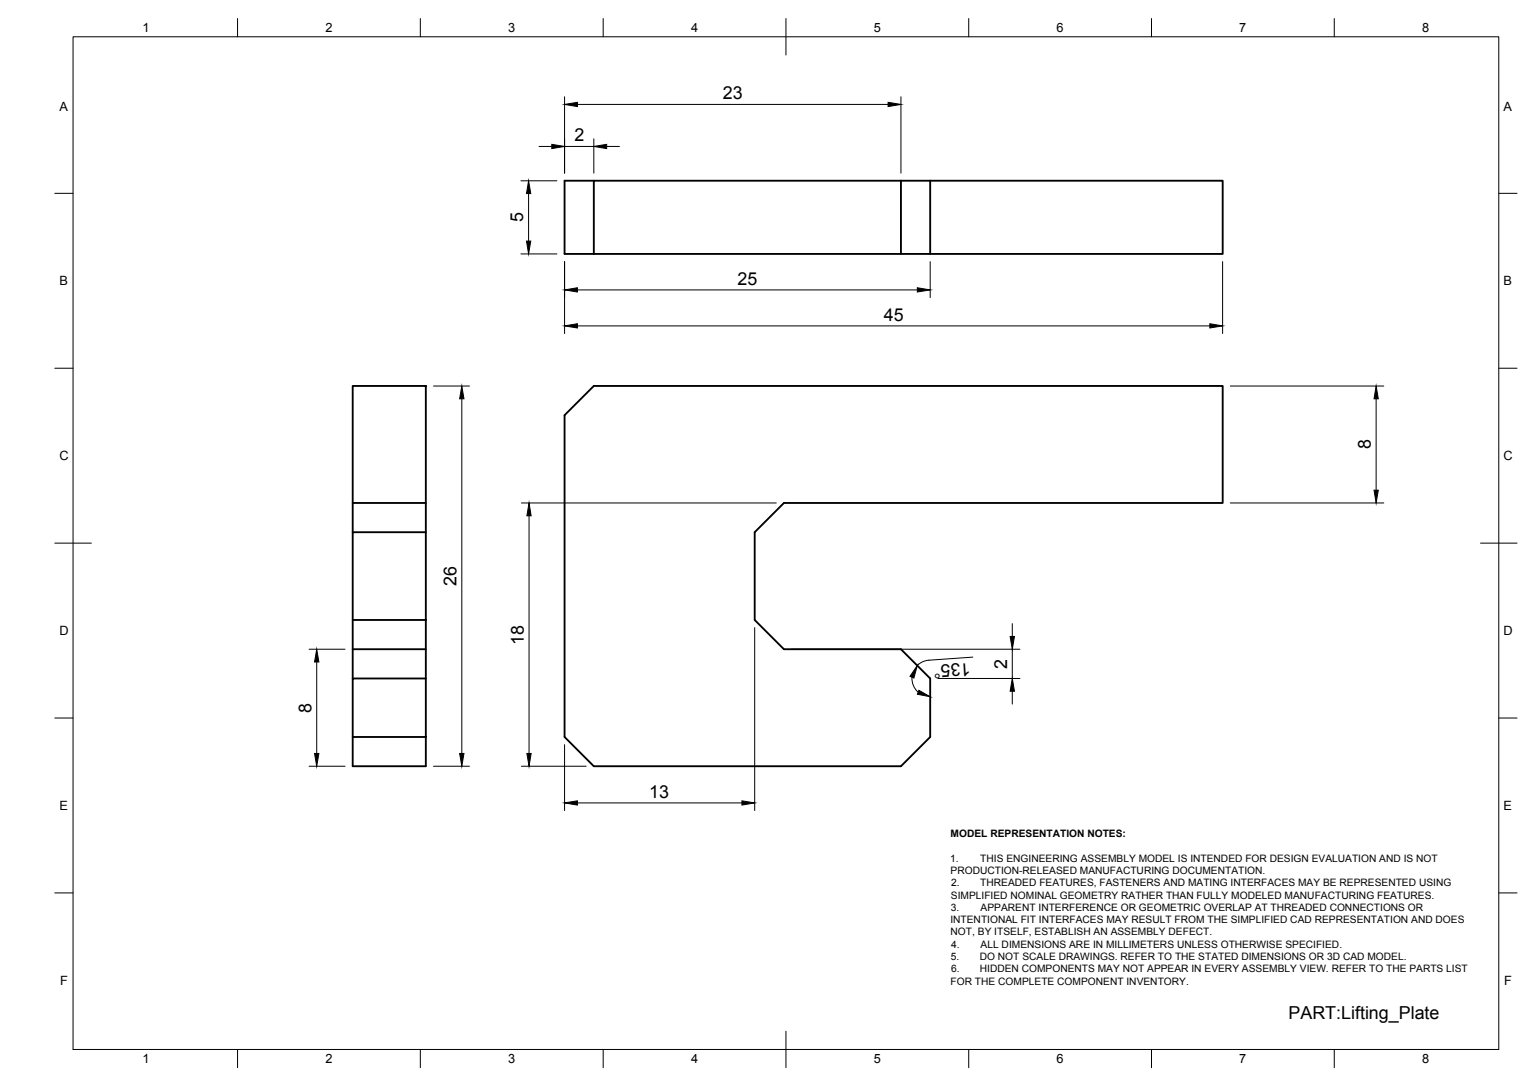
ISO-10303-21;
HEADER;
/* Generated by software containing ST-Developer
 * from STEP Tools, Inc. (www.steptools.com) 
 */

FILE_DESCRIPTION(
/* description */ ('STEP AP214'),
/* implementation_level */ '2;1');

FILE_NAME(
/* name */ 'Lifting_Plate.step',
/* time_stamp */ '2026-10-05T13:15:56-07:00',
/* author */ (''),
/* organization */ (''),
/* preprocessor_version */ 'ST-DEVELOPER v20.2',
/* originating_system */ 'Autodesk Translation Framework v15.15.0.0',
/* authorisation */ '');

FILE_SCHEMA (('AUTOMOTIVE_DESIGN { 1 0 10303 214 3 1 1 }'));
ENDSEC;

DATA;
#10=MECHANICAL_DESIGN_GEOMETRIC_PRESENTATION_REPRESENTATION('',(#1355),#37881);
#1331=SHAPE_REPRESENTATION_RELATIONSHIP('SRR','None',#37964,#1343);
#1343=ADVANCED_BREP_SHAPE_REPRESENTATION('',(#1367),#37879);
#1355=STYLED_ITEM('',(#38023),#1367);
#1367=MANIFOLD_SOLID_BREP('Body1',#10829);
#1547=PLANE('',#11824);
#1548=PLANE('',#11825);
#1549=PLANE('',#11826);
#1550=PLANE('',#11827);
#1551=PLANE('',#11828);
#1552=PLANE('',#11829);
#1553=PLANE('',#11830);
#1554=PLANE('',#11831);
#1555=PLANE('',#11832);
#1556=PLANE('',#11833);
#1557=PLANE('',#11834);
#1558=PLANE('',#11835);
#1559=PLANE('',#11836);
#1560=PLANE('',#11837);
#1561=PLANE('',#11838);
#1562=PLANE('',#11839);
#2154=FACE_OUTER_BOUND('',#2849,.T.);
#2155=FACE_OUTER_BOUND('',#2850,.T.);
#2156=FACE_OUTER_BOUND('',#2851,.T.);
#2157=FACE_OUTER_BOUND('',#2852,.T.);
#2158=FACE_OUTER_BOUND('',#2853,.T.);
#2159=FACE_OUTER_BOUND('',#2854,.T.);
#2160=FACE_OUTER_BOUND('',#2855,.T.);
#2161=FACE_OUTER_BOUND('',#2856,.T.);
#2162=FACE_OUTER_BOUND('',#2857,.T.);
#2163=FACE_OUTER_BOUND('',#2858,.T.);
#2164=FACE_OUTER_BOUND('',#2859,.T.);
#2165=FACE_OUTER_BOUND('',#2860,.T.);
#2166=FACE_OUTER_BOUND('',#2861,.T.);
#2167=FACE_OUTER_BOUND('',#2862,.T.);
#2168=FACE_OUTER_BOUND('',#2863,.T.);
#2169=FACE_OUTER_BOUND('',#2864,.T.);
#2849=EDGE_LOOP('',(#9933,#9934,#9935,#9936));
#2850=EDGE_LOOP('',(#9937,#9938,#9939,#9940));
#2851=EDGE_LOOP('',(#9941,#9942,#9943,#9944));
#2852=EDGE_LOOP('',(#9945,#9946,#9947,#9948));
#2853=EDGE_LOOP('',(#9949,#9950,#9951,#9952));
#2854=EDGE_LOOP('',(#9953,#9954,#9955,#9956));
#2855=EDGE_LOOP('',(#9957,#9958,#9959,#9960));
#2856=EDGE_LOOP('',(#9961,#9962,#9963,#9964));
#2857=EDGE_LOOP('',(#9965,#9966,#9967,#9968,#9969,#9970,#9971,#9972,#9973,
#9974,#9975,#9976,#9977,#9978));
#2858=EDGE_LOOP('',(#9979,#9980,#9981,#9982,#9983,#9984,#9985,#9986,#9987,
#9988,#9989,#9990,#9991,#9992));
#2859=EDGE_LOOP('',(#9993,#9994,#9995,#9996));
#2860=EDGE_LOOP('',(#9997,#9998,#9999,#10000));
#2861=EDGE_LOOP('',(#10001,#10002,#10003,#10004));
#2862=EDGE_LOOP('',(#10005,#10006,#10007,#10008));
#2863=EDGE_LOOP('',(#10009,#10010,#10011,#10012));
#2864=EDGE_LOOP('',(#10013,#10014,#10015,#10016));
#3128=LINE('',#37715,#3429);
#3129=LINE('',#37717,#3430);
#3130=LINE('',#37719,#3431);
#3131=LINE('',#37720,#3432);
#3132=LINE('',#37724,#3433);
#3133=LINE('',#37726,#3434);
#3134=LINE('',#37728,#3435);
#3135=LINE('',#37729,#3436);
#3136=LINE('',#37733,#3437);
#3137=LINE('',#37735,#3438);
#3138=LINE('',#37737,#3439);
#3139=LINE('',#37738,#3440);
#3140=LINE('',#37742,#3441);
#3141=LINE('',#37744,#3442);
#3142=LINE('',#37746,#3443);
#3143=LINE('',#37747,#3444);
#3144=LINE('',#37750,#3445);
#3145=LINE('',#37752,#3446);
#3146=LINE('',#37753,#3447);
#3147=LINE('',#37756,#3448);
#3148=LINE('',#37758,#3449);
#3149=LINE('',#37759,#3450);
#3150=LINE('',#37763,#3451);
#3151=LINE('',#37765,#3452);
#3152=LINE('',#37767,#3453);
#3153=LINE('',#37768,#3454);
#3154=LINE('',#37772,#3455);
#3155=LINE('',#37774,#3456);
#3156=LINE('',#37776,#3457);
#3157=LINE('',#37777,#3458);
#3158=LINE('',#37779,#3459);
#3159=LINE('',#37780,#3460);
#3160=LINE('',#37781,#3461);
#3161=LINE('',#37782,#3462);
#3162=LINE('',#37783,#3463);
#3163=LINE('',#37784,#3464);
#3164=LINE('',#37786,#3465);
#3165=LINE('',#37787,#3466);
#3166=LINE('',#37788,#3467);
#3167=LINE('',#37789,#3468);
#3168=LINE('',#37790,#3469);
#3169=LINE('',#37791,#3470);
#3429=VECTOR('',#13869,1000.);
#3430=VECTOR('',#13870,1000.);
#3431=VECTOR('',#13871,1000.);
#3432=VECTOR('',#13872,1000.);
#3433=VECTOR('',#13875,1000.);
#3434=VECTOR('',#13876,1000.);
#3435=VECTOR('',#13877,1000.);
#3436=VECTOR('',#13878,1000.);
#3437=VECTOR('',#13881,1000.);
#3438=VECTOR('',#13882,1000.);
#3439=VECTOR('',#13883,1000.);
#3440=VECTOR('',#13884,1000.);
#3441=VECTOR('',#13887,1000.);
#3442=VECTOR('',#13888,1000.);
#3443=VECTOR('',#13889,1000.);
#3444=VECTOR('',#13890,1000.);
#3445=VECTOR('',#13893,1000.);
#3446=VECTOR('',#13894,1000.);
#3447=VECTOR('',#13895,1000.);
#3448=VECTOR('',#13898,1000.);
#3449=VECTOR('',#13899,1000.);
#3450=VECTOR('',#13900,1000.);
#3451=VECTOR('',#13903,1000.);
#3452=VECTOR('',#13904,1000.);
#3453=VECTOR('',#13905,1000.);
#3454=VECTOR('',#13906,1000.);
#3455=VECTOR('',#13909,1000.);
#3456=VECTOR('',#13910,1000.);
#3457=VECTOR('',#13911,1000.);
#3458=VECTOR('',#13912,1000.);
#3459=VECTOR('',#13915,1000.);
#3460=VECTOR('',#13916,1000.);
#3461=VECTOR('',#13917,1000.);
#3462=VECTOR('',#13918,1000.);
#3463=VECTOR('',#13919,1000.);
#3464=VECTOR('',#13920,1000.);
#3465=VECTOR('',#13923,1000.);
#3466=VECTOR('',#13924,1000.);
#3467=VECTOR('',#13925,1000.);
#3468=VECTOR('',#13926,1000.);
#3469=VECTOR('',#13927,1000.);
#3470=VECTOR('',#13928,1000.);
#5041=VERTEX_POINT('',#37713);
#5042=VERTEX_POINT('',#37714);
#5043=VERTEX_POINT('',#37716);
#5044=VERTEX_POINT('',#37718);
#5045=VERTEX_POINT('',#37722);
#5046=VERTEX_POINT('',#37723);
#5047=VERTEX_POINT('',#37725);
#5048=VERTEX_POINT('',#37727);
#5049=VERTEX_POINT('',#37731);
#5050=VERTEX_POINT('',#37732);
#5051=VERTEX_POINT('',#37734);
#5052=VERTEX_POINT('',#37736);
#5053=VERTEX_POINT('',#37740);
#5054=VERTEX_POINT('',#37741);
#5055=VERTEX_POINT('',#37743);
#5056=VERTEX_POINT('',#37745);
#5057=VERTEX_POINT('',#37749);
#5058=VERTEX_POINT('',#37751);
#5059=VERTEX_POINT('',#37755);
#5060=VERTEX_POINT('',#37757);
#5061=VERTEX_POINT('',#37761);
#5062=VERTEX_POINT('',#37762);
#5063=VERTEX_POINT('',#37764);
#5064=VERTEX_POINT('',#37766);
#5065=VERTEX_POINT('',#37770);
#5066=VERTEX_POINT('',#37771);
#5067=VERTEX_POINT('',#37773);
#5068=VERTEX_POINT('',#37775);
#6677=EDGE_CURVE('',#5041,#5042,#3128,.T.);
#6678=EDGE_CURVE('',#5042,#5043,#3129,.T.);
#6679=EDGE_CURVE('',#5044,#5043,#3130,.T.);
#6680=EDGE_CURVE('',#5044,#5041,#3131,.T.);
#6681=EDGE_CURVE('',#5045,#5046,#3132,.T.);
#6682=EDGE_CURVE('',#5045,#5047,#3133,.T.);
#6683=EDGE_CURVE('',#5047,#5048,#3134,.T.);
#6684=EDGE_CURVE('',#5048,#5046,#3135,.T.);
#6685=EDGE_CURVE('',#5049,#5050,#3136,.T.);
#6686=EDGE_CURVE('',#5049,#5051,#3137,.T.);
#6687=EDGE_CURVE('',#5051,#5052,#3138,.T.);
#6688=EDGE_CURVE('',#5052,#5050,#3139,.T.);
#6689=EDGE_CURVE('',#5053,#5054,#3140,.T.);
#6690=EDGE_CURVE('',#5054,#5055,#3141,.T.);
#6691=EDGE_CURVE('',#5056,#5055,#3142,.T.);
#6692=EDGE_CURVE('',#5053,#5056,#3143,.T.);
#6693=EDGE_CURVE('',#5057,#5056,#3144,.T.);
#6694=EDGE_CURVE('',#5058,#5057,#3145,.T.);
#6695=EDGE_CURVE('',#5058,#5053,#3146,.T.);
#6696=EDGE_CURVE('',#5059,#5057,#3147,.T.);
#6697=EDGE_CURVE('',#5059,#5060,#3148,.T.);
#6698=EDGE_CURVE('',#5060,#5058,#3149,.T.);
#6699=EDGE_CURVE('',#5061,#5062,#3150,.T.);
#6700=EDGE_CURVE('',#5062,#5063,#3151,.T.);
#6701=EDGE_CURVE('',#5064,#5063,#3152,.T.);
#6702=EDGE_CURVE('',#5064,#5061,#3153,.T.);
#6703=EDGE_CURVE('',#5065,#5066,#3154,.T.);
#6704=EDGE_CURVE('',#5066,#5067,#3155,.T.);
#6705=EDGE_CURVE('',#5068,#5067,#3156,.T.);
#6706=EDGE_CURVE('',#5068,#5065,#3157,.T.);
#6707=EDGE_CURVE('',#5051,#5054,#3158,.T.);
#6708=EDGE_CURVE('',#5060,#5062,#3159,.T.);
#6709=EDGE_CURVE('',#5061,#5066,#3160,.T.);
#6710=EDGE_CURVE('',#5065,#5042,#3161,.T.);
#6711=EDGE_CURVE('',#5041,#5048,#3162,.T.);
#6712=EDGE_CURVE('',#5047,#5052,#3163,.T.);
#6713=EDGE_CURVE('',#5055,#5049,#3164,.T.);
#6714=EDGE_CURVE('',#5050,#5045,#3165,.T.);
#6715=EDGE_CURVE('',#5046,#5044,#3166,.T.);
#6716=EDGE_CURVE('',#5043,#5068,#3167,.T.);
#6717=EDGE_CURVE('',#5067,#5064,#3168,.T.);
#6718=EDGE_CURVE('',#5063,#5059,#3169,.T.);
#9933=ORIENTED_EDGE('',*,*,#6677,.T.);
#9934=ORIENTED_EDGE('',*,*,#6678,.T.);
#9935=ORIENTED_EDGE('',*,*,#6679,.F.);
#9936=ORIENTED_EDGE('',*,*,#6680,.T.);
#9937=ORIENTED_EDGE('',*,*,#6681,.F.);
#9938=ORIENTED_EDGE('',*,*,#6682,.T.);
#9939=ORIENTED_EDGE('',*,*,#6683,.T.);
#9940=ORIENTED_EDGE('',*,*,#6684,.T.);
#9941=ORIENTED_EDGE('',*,*,#6685,.F.);
#9942=ORIENTED_EDGE('',*,*,#6686,.T.);
#9943=ORIENTED_EDGE('',*,*,#6687,.T.);
#9944=ORIENTED_EDGE('',*,*,#6688,.T.);
#9945=ORIENTED_EDGE('',*,*,#6689,.T.);
#9946=ORIENTED_EDGE('',*,*,#6690,.T.);
#9947=ORIENTED_EDGE('',*,*,#6691,.F.);
#9948=ORIENTED_EDGE('',*,*,#6692,.F.);
#9949=ORIENTED_EDGE('',*,*,#6693,.F.);
#9950=ORIENTED_EDGE('',*,*,#6694,.F.);
#9951=ORIENTED_EDGE('',*,*,#6695,.T.);
#9952=ORIENTED_EDGE('',*,*,#6692,.T.);
#9953=ORIENTED_EDGE('',*,*,#6696,.F.);
#9954=ORIENTED_EDGE('',*,*,#6697,.T.);
#9955=ORIENTED_EDGE('',*,*,#6698,.T.);
#9956=ORIENTED_EDGE('',*,*,#6694,.T.);
#9957=ORIENTED_EDGE('',*,*,#6699,.T.);
#9958=ORIENTED_EDGE('',*,*,#6700,.T.);
#9959=ORIENTED_EDGE('',*,*,#6701,.F.);
#9960=ORIENTED_EDGE('',*,*,#6702,.T.);
#9961=ORIENTED_EDGE('',*,*,#6703,.T.);
#9962=ORIENTED_EDGE('',*,*,#6704,.T.);
#9963=ORIENTED_EDGE('',*,*,#6705,.F.);
#9964=ORIENTED_EDGE('',*,*,#6706,.T.);
#9965=ORIENTED_EDGE('',*,*,#6687,.F.);
#9966=ORIENTED_EDGE('',*,*,#6707,.T.);
#9967=ORIENTED_EDGE('',*,*,#6689,.F.);
#9968=ORIENTED_EDGE('',*,*,#6695,.F.);
#9969=ORIENTED_EDGE('',*,*,#6698,.F.);
#9970=ORIENTED_EDGE('',*,*,#6708,.T.);
#9971=ORIENTED_EDGE('',*,*,#6699,.F.);
#9972=ORIENTED_EDGE('',*,*,#6709,.T.);
#9973=ORIENTED_EDGE('',*,*,#6703,.F.);
#9974=ORIENTED_EDGE('',*,*,#6710,.T.);
#9975=ORIENTED_EDGE('',*,*,#6677,.F.);
#9976=ORIENTED_EDGE('',*,*,#6711,.T.);
#9977=ORIENTED_EDGE('',*,*,#6683,.F.);
#9978=ORIENTED_EDGE('',*,*,#6712,.T.);
#9979=ORIENTED_EDGE('',*,*,#6691,.T.);
#9980=ORIENTED_EDGE('',*,*,#6713,.T.);
#9981=ORIENTED_EDGE('',*,*,#6685,.T.);
#9982=ORIENTED_EDGE('',*,*,#6714,.T.);
#9983=ORIENTED_EDGE('',*,*,#6681,.T.);
#9984=ORIENTED_EDGE('',*,*,#6715,.T.);
#9985=ORIENTED_EDGE('',*,*,#6679,.T.);
#9986=ORIENTED_EDGE('',*,*,#6716,.T.);
#9987=ORIENTED_EDGE('',*,*,#6705,.T.);
#9988=ORIENTED_EDGE('',*,*,#6717,.T.);
#9989=ORIENTED_EDGE('',*,*,#6701,.T.);
#9990=ORIENTED_EDGE('',*,*,#6718,.T.);
#9991=ORIENTED_EDGE('',*,*,#6696,.T.);
#9992=ORIENTED_EDGE('',*,*,#6693,.T.);
#9993=ORIENTED_EDGE('',*,*,#6707,.F.);
#9994=ORIENTED_EDGE('',*,*,#6686,.F.);
#9995=ORIENTED_EDGE('',*,*,#6713,.F.);
#9996=ORIENTED_EDGE('',*,*,#6690,.F.);
#9997=ORIENTED_EDGE('',*,*,#6712,.F.);
#9998=ORIENTED_EDGE('',*,*,#6682,.F.);
#9999=ORIENTED_EDGE('',*,*,#6714,.F.);
#10000=ORIENTED_EDGE('',*,*,#6688,.F.);
#10001=ORIENTED_EDGE('',*,*,#6708,.F.);
#10002=ORIENTED_EDGE('',*,*,#6697,.F.);
#10003=ORIENTED_EDGE('',*,*,#6718,.F.);
#10004=ORIENTED_EDGE('',*,*,#6700,.F.);
#10005=ORIENTED_EDGE('',*,*,#6709,.F.);
#10006=ORIENTED_EDGE('',*,*,#6702,.F.);
#10007=ORIENTED_EDGE('',*,*,#6717,.F.);
#10008=ORIENTED_EDGE('',*,*,#6704,.F.);
#10009=ORIENTED_EDGE('',*,*,#6710,.F.);
#10010=ORIENTED_EDGE('',*,*,#6706,.F.);
#10011=ORIENTED_EDGE('',*,*,#6716,.F.);
#10012=ORIENTED_EDGE('',*,*,#6678,.F.);
#10013=ORIENTED_EDGE('',*,*,#6711,.F.);
#10014=ORIENTED_EDGE('',*,*,#6680,.F.);
#10015=ORIENTED_EDGE('',*,*,#6715,.F.);
#10016=ORIENTED_EDGE('',*,*,#6684,.F.);
#10799=ADVANCED_FACE('',(#2154),#1547,.T.);
#10800=ADVANCED_FACE('',(#2155),#1548,.T.);
#10801=ADVANCED_FACE('',(#2156),#1549,.T.);
#10802=ADVANCED_FACE('',(#2157),#1550,.T.);
#10803=ADVANCED_FACE('',(#2158),#1551,.T.);
#10804=ADVANCED_FACE('',(#2159),#1552,.T.);
#10805=ADVANCED_FACE('',(#2160),#1553,.T.);
#10806=ADVANCED_FACE('',(#2161),#1554,.T.);
#10807=ADVANCED_FACE('',(#2162),#1555,.T.);
#10808=ADVANCED_FACE('',(#2163),#1556,.F.);
#10809=ADVANCED_FACE('',(#2164),#1557,.F.);
#10810=ADVANCED_FACE('',(#2165),#1558,.F.);
#10811=ADVANCED_FACE('',(#2166),#1559,.T.);
#10812=ADVANCED_FACE('',(#2167),#1560,.T.);
#10813=ADVANCED_FACE('',(#2168),#1561,.F.);
#10814=ADVANCED_FACE('',(#2169),#1562,.F.);
#10829=CLOSED_SHELL('',(#10799,#10800,#10801,#10802,#10803,#10804,#10805,
#10806,#10807,#10808,#10809,#10810,#10811,#10812,#10813,#10814));
#11823=AXIS2_PLACEMENT_3D('',#37711,#13865,#13866);
#11824=AXIS2_PLACEMENT_3D('',#37712,#13867,#13868);
#11825=AXIS2_PLACEMENT_3D('',#37721,#13873,#13874);
#11826=AXIS2_PLACEMENT_3D('',#37730,#13879,#13880);
#11827=AXIS2_PLACEMENT_3D('',#37739,#13885,#13886);
#11828=AXIS2_PLACEMENT_3D('',#37748,#13891,#13892);
#11829=AXIS2_PLACEMENT_3D('',#37754,#13896,#13897);
#11830=AXIS2_PLACEMENT_3D('',#37760,#13901,#13902);
#11831=AXIS2_PLACEMENT_3D('',#37769,#13907,#13908);
#11832=AXIS2_PLACEMENT_3D('',#37778,#13913,#13914);
#11833=AXIS2_PLACEMENT_3D('',#37785,#13921,#13922);
#11834=AXIS2_PLACEMENT_3D('',#37792,#13929,#13930);
#11835=AXIS2_PLACEMENT_3D('',#37793,#13931,#13932);
#11836=AXIS2_PLACEMENT_3D('',#37794,#13933,#13934);
#11837=AXIS2_PLACEMENT_3D('',#37795,#13935,#13936);
#11838=AXIS2_PLACEMENT_3D('',#37796,#13937,#13938);
#11839=AXIS2_PLACEMENT_3D('',#37797,#13939,#13940);
#13865=DIRECTION('axis',(0.,0.,1.));
#13866=DIRECTION('refdir',(1.,0.,0.));
#13867=DIRECTION('center_axis',(0.,-1.,0.));
#13868=DIRECTION('ref_axis',(0.,0.,-1.));
#13869=DIRECTION('',(1.,0.,0.));
#13870=DIRECTION('',(0.,0.,1.));
#13871=DIRECTION('',(1.,0.,0.));
#13872=DIRECTION('',(0.,0.,-1.));
#13873=DIRECTION('center_axis',(-1.,0.,0.));
#13874=DIRECTION('ref_axis',(0.,0.,1.));
#13875=DIRECTION('',(0.,-1.,0.));
#13876=DIRECTION('',(0.,0.,-1.));
#13877=DIRECTION('',(0.,-1.,0.));
#13878=DIRECTION('',(0.,0.,1.));
#13879=DIRECTION('center_axis',(0.,1.,0.));
#13880=DIRECTION('ref_axis',(0.,0.,1.));
#13881=DIRECTION('',(-1.,0.,0.));
#13882=DIRECTION('',(0.,0.,-1.));
#13883=DIRECTION('',(-1.,0.,0.));
#13884=DIRECTION('',(0.,0.,1.));
#13885=DIRECTION('center_axis',(1.,7.70988211545248E-17,0.));
#13886=DIRECTION('ref_axis',(-7.70988211545248E-17,1.,0.));
#13887=DIRECTION('',(-7.70988211545248E-17,1.,0.));
#13888=DIRECTION('',(0.,0.,1.));
#13889=DIRECTION('',(-7.70988211545248E-17,1.,0.));
#13890=DIRECTION('',(0.,0.,1.));
#13891=DIRECTION('center_axis',(4.33680868994202E-16,-1.,0.));
#13892=DIRECTION('ref_axis',(1.,4.33680868994202E-16,0.));
#13893=DIRECTION('',(1.,4.33680868994202E-16,0.));
#13894=DIRECTION('',(0.,0.,1.));
#13895=DIRECTION('',(1.,4.33680868994202E-16,0.));
#13896=DIRECTION('center_axis',(-1.,0.,0.));
#13897=DIRECTION('ref_axis',(0.,0.,1.));
#13898=DIRECTION('',(0.,-1.,0.));
#13899=DIRECTION('',(0.,0.,-1.));
#13900=DIRECTION('',(0.,-1.,0.));
#13901=DIRECTION('center_axis',(1.73472347597681E-16,-1.,0.));
#13902=DIRECTION('ref_axis',(1.,1.73472347597681E-16,0.));
#13903=DIRECTION('',(1.,1.73472347597681E-16,0.));
#13904=DIRECTION('',(0.,0.,1.));
#13905=DIRECTION('',(1.,1.73472347597681E-16,0.));
#13906=DIRECTION('',(0.,0.,-1.));
#13907=DIRECTION('center_axis',(1.,1.44560289664734E-16,0.));
#13908=DIRECTION('ref_axis',(-1.44560289664734E-16,1.,0.));
#13909=DIRECTION('',(-1.44560289664734E-16,1.,0.));
#13910=DIRECTION('',(0.,0.,1.));
#13911=DIRECTION('',(-1.44560289664734E-16,1.,0.));
#13912=DIRECTION('',(0.,0.,-1.));
#13913=DIRECTION('center_axis',(0.,0.,-1.));
#13914=DIRECTION('ref_axis',(-1.,0.,0.));
#13915=DIRECTION('',(0.707106781186549,-0.707106781186546,0.));
#13916=DIRECTION('',(-0.707106781186551,0.707106781186544,0.));
#13917=DIRECTION('',(-0.707106781186545,-0.70710678118655,0.));
#13918=DIRECTION('',(-0.707106781186545,-0.70710678118655,0.));
#13919=DIRECTION('',(-0.70710678118655,0.707106781186545,0.));
#13920=DIRECTION('',(0.707106781186545,0.70710678118655,0.));
#13921=DIRECTION('center_axis',(0.,0.,-1.));
#13922=DIRECTION('ref_axis',(-1.,0.,0.));
#13923=DIRECTION('',(-0.707106781186549,0.707106781186546,0.));
#13924=DIRECTION('',(-0.707106781186545,-0.70710678118655,0.));
#13925=DIRECTION('',(0.70710678118655,-0.707106781186545,0.));
#13926=DIRECTION('',(0.707106781186545,0.70710678118655,0.));
#13927=DIRECTION('',(0.707106781186545,0.70710678118655,0.));
#13928=DIRECTION('',(0.707106781186551,-0.707106781186544,0.));
#13929=DIRECTION('center_axis',(-0.707106781186546,-0.707106781186549,0.));
#13930=DIRECTION('ref_axis',(0.,0.,1.));
#13931=DIRECTION('center_axis',(0.70710678118655,-0.707106781186545,0.));
#13932=DIRECTION('ref_axis',(0.,0.,1.));
#13933=DIRECTION('center_axis',(-0.707106781186544,-0.707106781186551,0.));
#13934=DIRECTION('ref_axis',(0.,0.,-1.));
#13935=DIRECTION('center_axis',(0.70710678118655,-0.707106781186545,0.));
#13936=DIRECTION('ref_axis',(0.,0.,-1.));
#13937=DIRECTION('center_axis',(-0.70710678118655,0.707106781186545,0.));
#13938=DIRECTION('ref_axis',(0.,0.,1.));
#13939=DIRECTION('center_axis',(0.707106781186545,0.70710678118655,0.));
#13940=DIRECTION('ref_axis',(0.,0.,1.));
#37711=CARTESIAN_POINT('',(0.,0.,0.));
#37712=CARTESIAN_POINT('Origin',(8.,0.,-5.));
#37713=CARTESIAN_POINT('',(2.00000000000001,0.,-5.));
#37714=CARTESIAN_POINT('',(6.00000000000001,0.,-5.));
#37715=CARTESIAN_POINT('',(8.,0.,-5.));
#37716=CARTESIAN_POINT('',(6.00000000000001,0.,0.));
#37717=CARTESIAN_POINT('',(6.00000000000001,0.,-5.));
#37718=CARTESIAN_POINT('',(2.00000000000001,0.,0.));
#37719=CARTESIAN_POINT('',(8.,0.,0.));
#37720=CARTESIAN_POINT('',(2.00000000000001,0.,-5.));
#37721=CARTESIAN_POINT('Origin',(0.,0.,-5.));
#37722=CARTESIAN_POINT('',(0.,23.,0.));
#37723=CARTESIAN_POINT('',(0.,2.,0.));
#37724=CARTESIAN_POINT('',(0.,0.,0.));
#37725=CARTESIAN_POINT('',(0.,23.,-5.));
#37726=CARTESIAN_POINT('',(0.,23.,-5.));
#37727=CARTESIAN_POINT('',(0.,2.,-5.));
#37728=CARTESIAN_POINT('',(0.,0.,-5.));
#37729=CARTESIAN_POINT('',(0.,2.,-5.));
#37730=CARTESIAN_POINT('Origin',(0.,25.,-5.));
#37731=CARTESIAN_POINT('',(24.,25.,0.));
#37732=CARTESIAN_POINT('',(2.,25.,0.));
#37733=CARTESIAN_POINT('',(0.,25.,0.));
#37734=CARTESIAN_POINT('',(24.,25.,-5.));
#37735=CARTESIAN_POINT('',(24.,25.,-5.));
#37736=CARTESIAN_POINT('',(2.,25.,-5.));
#37737=CARTESIAN_POINT('',(0.,25.,-5.));
#37738=CARTESIAN_POINT('',(2.,25.,-5.));
#37739=CARTESIAN_POINT('Origin',(26.,25.,-5.));
#37740=CARTESIAN_POINT('',(26.,-20.,-5.));
#37741=CARTESIAN_POINT('',(26.,23.,-5.));
#37742=CARTESIAN_POINT('',(26.,25.,-5.));
#37743=CARTESIAN_POINT('',(26.,23.,0.));
#37744=CARTESIAN_POINT('',(26.,23.,-5.));
#37745=CARTESIAN_POINT('',(26.,-20.,0.));
#37746=CARTESIAN_POINT('',(26.,25.,0.));
#37747=CARTESIAN_POINT('',(26.,-20.,-5.));
#37748=CARTESIAN_POINT('Origin',(26.,-20.,-5.));
#37749=CARTESIAN_POINT('',(18.,-20.,0.));
#37750=CARTESIAN_POINT('',(26.,-20.,0.));
#37751=CARTESIAN_POINT('',(18.,-20.,-5.));
#37752=CARTESIAN_POINT('',(18.,-20.,-5.));
#37753=CARTESIAN_POINT('',(26.,-20.,-5.));
#37754=CARTESIAN_POINT('Origin',(18.,-20.,-5.));
#37755=CARTESIAN_POINT('',(18.,10.,0.));
#37756=CARTESIAN_POINT('',(18.,-20.,0.));
#37757=CARTESIAN_POINT('',(18.,10.,-5.));
#37758=CARTESIAN_POINT('',(18.,10.,-5.));
#37759=CARTESIAN_POINT('',(18.,-20.,-5.));
#37760=CARTESIAN_POINT('Origin',(18.,12.,-5.));
#37761=CARTESIAN_POINT('',(10.,12.,-5.));
#37762=CARTESIAN_POINT('',(16.,12.,-5.));
#37763=CARTESIAN_POINT('',(18.,12.,-5.));
#37764=CARTESIAN_POINT('',(16.,12.,0.));
#37765=CARTESIAN_POINT('',(16.,12.,0.));
#37766=CARTESIAN_POINT('',(10.,12.,0.));
#37767=CARTESIAN_POINT('',(18.,12.,0.));
#37768=CARTESIAN_POINT('',(10.,12.,-5.));
#37769=CARTESIAN_POINT('Origin',(8.,12.,-5.));
#37770=CARTESIAN_POINT('',(8.,2.,-5.));
#37771=CARTESIAN_POINT('',(8.,9.99999999999998,-5.));
#37772=CARTESIAN_POINT('',(8.,12.,-5.));
#37773=CARTESIAN_POINT('',(8.,9.99999999999998,0.));
#37774=CARTESIAN_POINT('',(8.,9.99999999999998,0.));
#37775=CARTESIAN_POINT('',(8.,2.,0.));
#37776=CARTESIAN_POINT('',(8.,12.,0.));
#37777=CARTESIAN_POINT('',(8.,2.,-5.));
#37778=CARTESIAN_POINT('Origin',(0.,0.,-5.));
#37779=CARTESIAN_POINT('',(24.5,24.5,-5.));
#37780=CARTESIAN_POINT('',(16.,12.,-5.));
#37781=CARTESIAN_POINT('',(8.,9.99999999999998,-5.));
#37782=CARTESIAN_POINT('',(3.00000000000003,-3.00000000000001,-5.));
#37783=CARTESIAN_POINT('',(0.999999999999998,1.,-5.));
#37784=CARTESIAN_POINT('',(-11.5,11.4999999999999,-5.));
#37785=CARTESIAN_POINT('Origin',(0.,0.,0.));
#37786=CARTESIAN_POINT('',(26.,23.,0.));
#37787=CARTESIAN_POINT('',(2.,25.,0.));
#37788=CARTESIAN_POINT('',(0.,2.,0.));
#37789=CARTESIAN_POINT('',(6.00000000000001,0.,0.));
#37790=CARTESIAN_POINT('',(-0.999999999999961,0.999999999999954,0.));
#37791=CARTESIAN_POINT('',(13.9999999999999,14.0000000000001,0.));
#37792=CARTESIAN_POINT('Origin',(26.,23.,-5.));
#37793=CARTESIAN_POINT('Origin',(2.,25.,-5.));
#37794=CARTESIAN_POINT('Origin',(16.,12.,-5.));
#37795=CARTESIAN_POINT('Origin',(8.,9.99999999999998,-5.));
#37796=CARTESIAN_POINT('Origin',(6.00000000000001,0.,-5.));
#37797=CARTESIAN_POINT('Origin',(0.,2.,-5.));
#37865=UNCERTAINTY_MEASURE_WITH_UNIT(LENGTH_MEASURE(0.01),#37882,
'DISTANCE_ACCURACY_VALUE',
'Maximum model space distance between geometric entities at asserted c
onnectivities');
#37867=UNCERTAINTY_MEASURE_WITH_UNIT(LENGTH_MEASURE(0.01),#37882,
'DISTANCE_ACCURACY_VALUE',
'Maximum model space distance between geometric entities at asserted c
onnectivities');
#37879=(
GEOMETRIC_REPRESENTATION_CONTEXT(3)
GLOBAL_UNCERTAINTY_ASSIGNED_CONTEXT((#37865))
GLOBAL_UNIT_ASSIGNED_CONTEXT((#37882,#37884,#37885))
REPRESENTATION_CONTEXT('','3D')
);
#37881=(
GEOMETRIC_REPRESENTATION_CONTEXT(3)
GLOBAL_UNCERTAINTY_ASSIGNED_CONTEXT((#37867))
GLOBAL_UNIT_ASSIGNED_CONTEXT((#37882,#37884,#37885))
REPRESENTATION_CONTEXT('','3D')
);
#37882=(
LENGTH_UNIT()
NAMED_UNIT(*)
SI_UNIT(.MILLI.,.METRE.)
);
#37884=(
NAMED_UNIT(*)
PLANE_ANGLE_UNIT()
SI_UNIT($,.RADIAN.)
);
#37885=(
NAMED_UNIT(*)
SI_UNIT($,.STERADIAN.)
SOLID_ANGLE_UNIT()
);
#37897=SHAPE_DEFINITION_REPRESENTATION(#37910,#37964);
#37910=PRODUCT_DEFINITION_SHAPE('',$,#37978);
#37964=SHAPE_REPRESENTATION('',(#11823),#37879);
#37966=PRODUCT_DEFINITION_CONTEXT('part definition',#38007,'design');
#37978=PRODUCT_DEFINITION('PS09','Lifting_Plate',#37991,#37966);
#37991=PRODUCT_DEFINITION_FORMATION('',$,#38020);
#38007=APPLICATION_CONTEXT(
'Core Data for Automotive Mechanical Design Process');
#38008=PRODUCT_CONTEXT('part definition',#38007,'mechanical');
#38020=PRODUCT('PS09','Lifting_Plate',$,(#38008));
#38023=PRESENTATION_STYLE_ASSIGNMENT((#38025));
#38025=SURFACE_STYLE_USAGE(.BOTH.,#38027);
#38027=SURFACE_SIDE_STYLE('',(#38029));
#38029=SURFACE_STYLE_FILL_AREA(#38031);
#38031=FILL_AREA_STYLE('Opaque(202,209,238)',(#38033));
#38033=FILL_AREA_STYLE_COLOUR('Opaque(202,209,238)',#38035);
#38035=COLOUR_RGB('Opaque(202,209,238)', 0.66274510, 0.83137255, 0.94901961);
ENDSEC;
END-ISO-10303-21;
